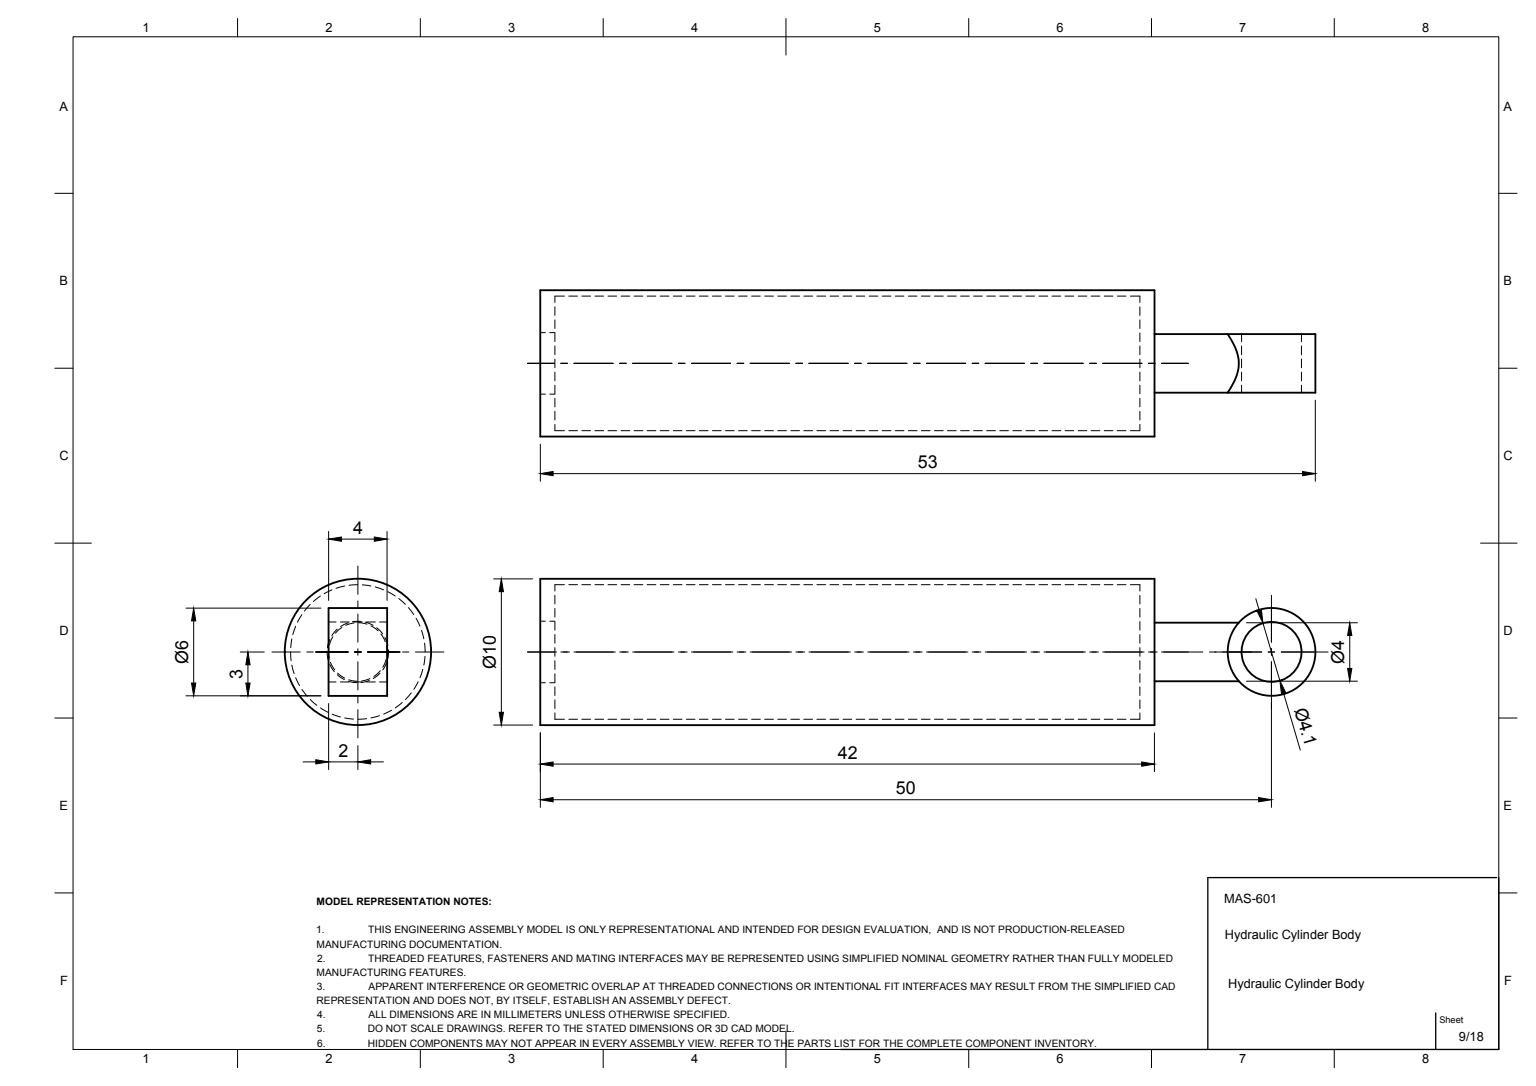
ISO-10303-21;
HEADER;
FILE_DESCRIPTION((''),'2;1');
FILE_NAME('Hydraulic Cylinder Body.step','2026-10-06T07:37:42+05:00',(''),(''),'','','');
FILE_SCHEMA (('AUTOMOTIVE_DESIGN { 1 0 10303 214 3 1 1 }'));
ENDSEC;
DATA;
#10=MECHANICAL_DESIGN_GEOMETRIC_PRESENTATION_REPRESENTATION('',(#377),#18757);
#343=SHAPE_REPRESENTATION_RELATIONSHIP('SRR','None',#18861,#360) ;
#360=ADVANCED_BREP_SHAPE_REPRESENTATION('',(#394),#18744) ;
#377=STYLED_ITEM('',(#18955),#394) ;
#394=MANIFOLD_SOLID_BREP('Hydraulic Cylinder Body',#9546) ;
#419=B_SPLINE_CURVE_WITH_KNOTS('',3,(#14585,#14586,#14587,#14588),
 .UNSPECIFIED.,.F.,.F.,(4,4),(0.941657228299601,0.974745769205032),
 .UNSPECIFIED.) ;
#420=B_SPLINE_CURVE_WITH_KNOTS('',3,(#14596,#14597,#14598,#14599,#14600,
#14601,#14602,#14603,#14604,#14605),.UNSPECIFIED.,.F.,.F.,(4,2,2,2,4),(0.313885742766534,
0.391923143756541,0.469960544746549,0.548866015139808,0.627771485533068),
 .UNSPECIFIED.) ;
#421=B_SPLINE_CURVE_WITH_KNOTS('',3,(#14606,#14607,#14608,#14609,#14610,
#14611,#14612,#14613,#14614,#14615),.UNSPECIFIED.,.F.,.F.,(4,2,2,2,4),(0.627771485533068,
0.706676955926327,0.785582426319586,0.863619827309594,0.941657228299601),
 .UNSPECIFIED.) ;
#422=B_SPLINE_CURVE_WITH_KNOTS('',3,(#14617,#14618,#14619,#14620,#14621,
#14622,#14623,#14624,#14625,#14626,#14627,#14628,#14629,#14630,#14631,#14632,
#14633,#14634,#14635),.UNSPECIFIED.,.F.,.F.,(4,2,2,2,3,2,2,2,4),(0.974745769205032,
1.01969462928961,1.09773203027962,1.17663750067288,1.25554297106614,1.33444844145939,
1.41335391185265,1.49139131284266,1.53634017292724),.UNSPECIFIED.) ;
#423=B_SPLINE_CURVE_WITH_KNOTS('',3,(#14667,#14668,#14669,#14670),
 .UNSPECIFIED.,.F.,.F.,(4,4),(1.53634017292724,1.56942871383267),
 .UNSPECIFIED.) ;
#561=CYLINDRICAL_SURFACE('',#10071,3.) ;
#562=CYLINDRICAL_SURFACE('',#10073,3.) ;
#563=CYLINDRICAL_SURFACE('',#10076,2.05) ;
#564=CYLINDRICAL_SURFACE('',#10081,4.6) ;
#565=CYLINDRICAL_SURFACE('',#10085,2.09999999999999) ;
#566=CYLINDRICAL_SURFACE('',#10089,4.99999999999999) ;
#567=CYLINDRICAL_SURFACE('',#10093,1.99999999999999) ;
#568=CYLINDRICAL_SURFACE('',#10094,3.) ;
#712=FACE_BOUND('',#1851,.T.) ;
#713=FACE_BOUND('',#1854,.T.) ;
#714=FACE_BOUND('',#1857,.T.) ;
#715=FACE_BOUND('',#1861,.T.) ;
#716=FACE_BOUND('',#1863,.T.) ;
#856=PLANE('',#10079) ;
#857=PLANE('',#10083) ;
#858=PLANE('',#10087) ;
#859=PLANE('',#10091) ;
#860=PLANE('',#10096) ;
#861=PLANE('',#10097) ;
#1265=FACE_OUTER_BOUND('',#1845,.T.) ;
#1266=FACE_OUTER_BOUND('',#1846,.T.) ;
#1267=FACE_OUTER_BOUND('',#1847,.T.) ;
#1268=FACE_OUTER_BOUND('',#1848,.T.) ;
#1269=FACE_OUTER_BOUND('',#1849,.T.) ;
#1270=FACE_OUTER_BOUND('',#1850,.T.) ;
#1271=FACE_OUTER_BOUND('',#1852,.T.) ;
#1272=FACE_OUTER_BOUND('',#1853,.T.) ;
#1273=FACE_OUTER_BOUND('',#1855,.T.) ;
#1274=FACE_OUTER_BOUND('',#1856,.T.) ;
#1275=FACE_OUTER_BOUND('',#1858,.T.) ;
#1276=FACE_OUTER_BOUND('',#1859,.T.) ;
#1277=FACE_OUTER_BOUND('',#1860,.T.) ;
#1278=FACE_OUTER_BOUND('',#1862,.T.) ;
#1845=EDGE_LOOP('',(#7257,#7258,#7259)) ;
#1846=EDGE_LOOP('',(#7260,#7261,#7262,#7263,#7264,#7265,#7266)) ;
#1847=EDGE_LOOP('',(#7267,#7268,#7269,#7270)) ;
#1848=EDGE_LOOP('',(#7271)) ;
#1849=EDGE_LOOP('',(#7272,#7273,#7274,#7275)) ;
#1850=EDGE_LOOP('',(#7276)) ;
#1851=EDGE_LOOP('',(#7277)) ;
#1852=EDGE_LOOP('',(#7278,#7279,#7280,#7281)) ;
#1853=EDGE_LOOP('',(#7282)) ;
#1854=EDGE_LOOP('',(#7283)) ;
#1855=EDGE_LOOP('',(#7284,#7285,#7286,#7287)) ;
#1856=EDGE_LOOP('',(#7288)) ;
#1857=EDGE_LOOP('',(#7289)) ;
#1858=EDGE_LOOP('',(#7290,#7291,#7292,#7293,#7294,#7295,#7296,#7297)) ;
#1859=EDGE_LOOP('',(#7298,#7299,#7300)) ;
#1860=EDGE_LOOP('',(#7301,#7302)) ;
#1861=EDGE_LOOP('',(#7303)) ;
#1862=EDGE_LOOP('',(#7304,#7305)) ;
#1863=EDGE_LOOP('',(#7306)) ;
#2538=LINE('',#14582,#3309) ;
#2539=LINE('',#14592,#3310) ;
#2540=LINE('',#14640,#3311) ;
#2541=LINE('',#14647,#3312) ;
#2542=LINE('',#14654,#3313) ;
#2543=LINE('',#14662,#3314) ;
#2544=LINE('',#14671,#3315) ;
#3309=VECTOR('',#11670,3.) ;
#3310=VECTOR('',#11675,3.) ;
#3311=VECTOR('',#11684,2.05) ;
#3312=VECTOR('',#11693,4.6) ;
#3313=VECTOR('',#11702,2.09999999999999) ;
#3314=VECTOR('',#11713,4.99999999999999) ;
#3315=VECTOR('',#11720,1.99999999999999) ;
#3915=CIRCLE('',#10072,3.) ;
#3916=CIRCLE('',#10074,3.) ;
#3917=CIRCLE('',#10075,3.) ;
#3918=CIRCLE('',#10077,2.05) ;
#3919=CIRCLE('',#10078,2.05) ;
#3920=CIRCLE('',#10080,4.6) ;
#3921=CIRCLE('',#10082,4.6) ;
#3922=CIRCLE('',#10084,2.1) ;
#3923=CIRCLE('',#10086,2.09999999999999) ;
#3924=CIRCLE('',#10088,4.99999999999999) ;
#3925=CIRCLE('',#10090,5.) ;
#3926=CIRCLE('',#10092,1.99999999999999) ;
#3927=CIRCLE('',#10095,3.) ;
#4450=VERTEX_POINT('',#14580) ;
#4451=VERTEX_POINT('',#14581) ;
#4452=VERTEX_POINT('',#14583) ;
#4453=VERTEX_POINT('',#14590) ;
#4454=VERTEX_POINT('',#14591) ;
#4455=VERTEX_POINT('',#14593) ;
#4456=VERTEX_POINT('',#14595) ;
#4457=VERTEX_POINT('',#14637) ;
#4458=VERTEX_POINT('',#14639) ;
#4459=VERTEX_POINT('',#14643) ;
#4460=VERTEX_POINT('',#14646) ;
#4461=VERTEX_POINT('',#14650) ;
#4462=VERTEX_POINT('',#14653) ;
#4463=VERTEX_POINT('',#14657) ;
#4464=VERTEX_POINT('',#14660) ;
#4465=VERTEX_POINT('',#14664) ;
#5475=EDGE_CURVE('',#4450,#4451,#2538,.T.) ;
#5476=EDGE_CURVE('',#4451,#4452,#3915,.T.) ;
#5477=EDGE_CURVE('',#4452,#4450,#419,.T.) ;
#5478=EDGE_CURVE('',#4453,#4454,#2539,.T.) ;
#5479=EDGE_CURVE('',#4455,#4453,#3916,.T.) ;
#5480=EDGE_CURVE('',#4455,#4456,#420,.T.) ;
#5481=EDGE_CURVE('',#4456,#4452,#421,.T.) ;
#5482=EDGE_CURVE('',#4452,#4451,#3917,.T.) ;
#5483=EDGE_CURVE('',#4450,#4454,#422,.T.) ;
#5484=EDGE_CURVE('',#4457,#4457,#3918,.T.) ;
#5485=EDGE_CURVE('',#4457,#4458,#2540,.T.) ;
#5486=EDGE_CURVE('',#4458,#4458,#3919,.T.) ;
#5487=EDGE_CURVE('',#4459,#4459,#3920,.T.) ;
#5488=EDGE_CURVE('',#4459,#4460,#2541,.T.) ;
#5489=EDGE_CURVE('',#4460,#4460,#3921,.T.) ;
#5490=EDGE_CURVE('',#4461,#4461,#3922,.T.) ;
#5491=EDGE_CURVE('',#4461,#4462,#2542,.T.) ;
#5492=EDGE_CURVE('',#4462,#4462,#3923,.T.) ;
#5493=EDGE_CURVE('',#4463,#4463,#3924,.T.) ;
#5494=EDGE_CURVE('',#4464,#4464,#3925,.T.) ;
#5495=EDGE_CURVE('',#4464,#4463,#2543,.T.) ;
#5496=EDGE_CURVE('',#4465,#4465,#3926,.T.) ;
#5497=EDGE_CURVE('',#4454,#4455,#423,.T.) ;
#5498=EDGE_CURVE('',#4456,#4465,#2544,.T.) ;
#5499=EDGE_CURVE('',#4453,#4455,#3927,.T.) ;
#7257=ORIENTED_EDGE('',*,*,#5475,.T.) ;
#7258=ORIENTED_EDGE('',*,*,#5476,.T.) ;
#7259=ORIENTED_EDGE('',*,*,#5477,.T.) ;
#7260=ORIENTED_EDGE('',*,*,#5478,.F.) ;
#7261=ORIENTED_EDGE('',*,*,#5479,.F.) ;
#7262=ORIENTED_EDGE('',*,*,#5480,.T.) ;
#7263=ORIENTED_EDGE('',*,*,#5481,.T.) ;
#7264=ORIENTED_EDGE('',*,*,#5482,.T.) ;
#7265=ORIENTED_EDGE('',*,*,#5475,.F.) ;
#7266=ORIENTED_EDGE('',*,*,#5483,.T.) ;
#7267=ORIENTED_EDGE('',*,*,#5484,.F.) ;
#7268=ORIENTED_EDGE('',*,*,#5485,.T.) ;
#7269=ORIENTED_EDGE('',*,*,#5486,.F.) ;
#7270=ORIENTED_EDGE('',*,*,#5485,.F.) ;
#7271=ORIENTED_EDGE('',*,*,#5487,.F.) ;
#7272=ORIENTED_EDGE('',*,*,#5487,.T.) ;
#7273=ORIENTED_EDGE('',*,*,#5488,.T.) ;
#7274=ORIENTED_EDGE('',*,*,#5489,.F.) ;
#7275=ORIENTED_EDGE('',*,*,#5488,.F.) ;
#7276=ORIENTED_EDGE('',*,*,#5489,.T.) ;
#7277=ORIENTED_EDGE('',*,*,#5490,.F.) ;
#7278=ORIENTED_EDGE('',*,*,#5490,.T.) ;
#7279=ORIENTED_EDGE('',*,*,#5491,.T.) ;
#7280=ORIENTED_EDGE('',*,*,#5492,.F.) ;
#7281=ORIENTED_EDGE('',*,*,#5491,.F.) ;
#7282=ORIENTED_EDGE('',*,*,#5493,.F.) ;
#7283=ORIENTED_EDGE('',*,*,#5492,.T.) ;
#7284=ORIENTED_EDGE('',*,*,#5494,.F.) ;
#7285=ORIENTED_EDGE('',*,*,#5495,.T.) ;
#7286=ORIENTED_EDGE('',*,*,#5493,.T.) ;
#7287=ORIENTED_EDGE('',*,*,#5495,.F.) ;
#7288=ORIENTED_EDGE('',*,*,#5494,.T.) ;
#7289=ORIENTED_EDGE('',*,*,#5496,.F.) ;
#7290=ORIENTED_EDGE('',*,*,#5480,.F.) ;
#7291=ORIENTED_EDGE('',*,*,#5497,.F.) ;
#7292=ORIENTED_EDGE('',*,*,#5483,.F.) ;
#7293=ORIENTED_EDGE('',*,*,#5477,.F.) ;
#7294=ORIENTED_EDGE('',*,*,#5481,.F.) ;
#7295=ORIENTED_EDGE('',*,*,#5498,.T.) ;
#7296=ORIENTED_EDGE('',*,*,#5496,.T.) ;
#7297=ORIENTED_EDGE('',*,*,#5498,.F.) ;
#7298=ORIENTED_EDGE('',*,*,#5478,.T.) ;
#7299=ORIENTED_EDGE('',*,*,#5497,.T.) ;
#7300=ORIENTED_EDGE('',*,*,#5499,.F.) ;
#7301=ORIENTED_EDGE('',*,*,#5479,.T.) ;
#7302=ORIENTED_EDGE('',*,*,#5499,.T.) ;
#7303=ORIENTED_EDGE('',*,*,#5486,.T.) ;
#7304=ORIENTED_EDGE('',*,*,#5482,.F.) ;
#7305=ORIENTED_EDGE('',*,*,#5476,.F.) ;
#7306=ORIENTED_EDGE('',*,*,#5484,.T.) ;
#9201=ADVANCED_FACE('',(#1265),#561,.T.) ;
#9202=ADVANCED_FACE('',(#1266),#562,.T.) ;
#9203=ADVANCED_FACE('',(#1267),#563,.F.) ;
#9204=ADVANCED_FACE('',(#1268),#856,.T.) ;
#9205=ADVANCED_FACE('',(#1269),#564,.F.) ;
#9206=ADVANCED_FACE('',(#1270,#712),#857,.T.) ;
#9207=ADVANCED_FACE('',(#1271),#565,.F.) ;
#9208=ADVANCED_FACE('',(#1272,#713),#858,.T.) ;
#9209=ADVANCED_FACE('',(#1273),#566,.T.) ;
#9210=ADVANCED_FACE('',(#1274,#714),#859,.T.) ;
#9211=ADVANCED_FACE('',(#1275),#567,.T.) ;
#9212=ADVANCED_FACE('',(#1276),#568,.T.) ;
#9213=ADVANCED_FACE('',(#1277,#715),#860,.T.) ;
#9214=ADVANCED_FACE('',(#1278,#716),#861,.F.) ;
#9546=CLOSED_SHELL('',(#9201,#9202,#9203,#9204,#9205,#9206,#9207,#9208,
#9209,#9210,#9211,#9212,#9213,#9214)) ;
#10070=AXIS2_PLACEMENT_3D('',#14578,#11666,#11667) ;
#10071=AXIS2_PLACEMENT_3D('',#14579,#11668,#11669) ;
#10072=AXIS2_PLACEMENT_3D('',#14584,#11671,#11672) ;
#10073=AXIS2_PLACEMENT_3D('',#14589,#11673,#11674) ;
#10074=AXIS2_PLACEMENT_3D('',#14594,#11676,#11677) ;
#10075=AXIS2_PLACEMENT_3D('',#14616,#11678,#11679) ;
#10076=AXIS2_PLACEMENT_3D('',#14636,#11680,#11681) ;
#10077=AXIS2_PLACEMENT_3D('',#14638,#11682,#11683) ;
#10078=AXIS2_PLACEMENT_3D('',#14641,#11685,#11686) ;
#10079=AXIS2_PLACEMENT_3D('',#14642,#11687,#11688) ;
#10080=AXIS2_PLACEMENT_3D('',#14644,#11689,#11690) ;
#10081=AXIS2_PLACEMENT_3D('',#14645,#11691,#11692) ;
#10082=AXIS2_PLACEMENT_3D('',#14648,#11694,#11695) ;
#10083=AXIS2_PLACEMENT_3D('',#14649,#11696,#11697) ;
#10084=AXIS2_PLACEMENT_3D('',#14651,#11698,#11699) ;
#10085=AXIS2_PLACEMENT_3D('',#14652,#11700,#11701) ;
#10086=AXIS2_PLACEMENT_3D('',#14655,#11703,#11704) ;
#10087=AXIS2_PLACEMENT_3D('',#14656,#11705,#11706) ;
#10088=AXIS2_PLACEMENT_3D('',#14658,#11707,#11708) ;
#10089=AXIS2_PLACEMENT_3D('',#14659,#11709,#11710) ;
#10090=AXIS2_PLACEMENT_3D('',#14661,#11711,#11712) ;
#10091=AXIS2_PLACEMENT_3D('',#14663,#11714,#11715) ;
#10092=AXIS2_PLACEMENT_3D('',#14665,#11716,#11717) ;
#10093=AXIS2_PLACEMENT_3D('',#14666,#11718,#11719) ;
#10094=AXIS2_PLACEMENT_3D('',#14672,#11721,#11722) ;
#10095=AXIS2_PLACEMENT_3D('',#14673,#11723,#11724) ;
#10096=AXIS2_PLACEMENT_3D('',#14674,#11725,#11726) ;
#10097=AXIS2_PLACEMENT_3D('',#14675,#11727,#11728) ;
#11666=DIRECTION('axis',(0.,0.,1.)) ;
#11667=DIRECTION('refdir',(1.,0.,0.)) ;
#11668=DIRECTION('center_axis',(0.,1.,0.)) ;
#11669=DIRECTION('ref_axis',(1.,0.,0.)) ;
#11670=DIRECTION('',(0.,-1.,0.)) ;
#11671=DIRECTION('center_axis',(0.,1.,0.)) ;
#11672=DIRECTION('ref_axis',(1.,0.,0.)) ;
#11673=DIRECTION('center_axis',(0.,1.,0.)) ;
#11674=DIRECTION('ref_axis',(1.,0.,0.)) ;
#11675=DIRECTION('',(0.,-1.,0.)) ;
#11676=DIRECTION('center_axis',(0.,1.,0.)) ;
#11677=DIRECTION('ref_axis',(1.,0.,0.)) ;
#11678=DIRECTION('center_axis',(0.,1.,0.)) ;
#11679=DIRECTION('ref_axis',(1.,0.,0.)) ;
#11680=DIRECTION('center_axis',(0.,1.,0.)) ;
#11681=DIRECTION('ref_axis',(1.,0.,0.)) ;
#11682=DIRECTION('center_axis',(0.,1.,0.)) ;
#11683=DIRECTION('ref_axis',(1.,0.,0.)) ;
#11684=DIRECTION('',(0.,1.,0.)) ;
#11685=DIRECTION('center_axis',(0.,-1.,0.)) ;
#11686=DIRECTION('ref_axis',(1.,0.,0.)) ;
#11687=DIRECTION('center_axis',(-0.993765553407216,0.,0.11149002135281)) ;
#11688=DIRECTION('ref_axis',(0.11149002135281,0.,0.993765553407216)) ;
#11689=DIRECTION('center_axis',(0.993765553407216,0.,-0.11149002135281)) ;
#11690=DIRECTION('ref_axis',(0.11149002135281,0.,0.993765553407216)) ;
#11691=DIRECTION('center_axis',(0.993765553407216,0.,-0.11149002135281)) ;
#11692=DIRECTION('ref_axis',(-0.111490021352808,0.,-0.993765553407216)) ;
#11693=DIRECTION('',(-0.993765553407216,0.,0.11149002135281)) ;
#11694=DIRECTION('center_axis',(0.993765553407216,0.,-0.11149002135281)) ;
#11695=DIRECTION('ref_axis',(0.11149002135281,0.,0.993765553407216)) ;
#11696=DIRECTION('center_axis',(0.993765553407216,0.,-0.11149002135281)) ;
#11697=DIRECTION('ref_axis',(-0.11149002135281,0.,-0.993765553407216)) ;
#11698=DIRECTION('center_axis',(0.993765553407216,0.,-0.11149002135281)) ;
#11699=DIRECTION('ref_axis',(0.11149002135281,0.,0.993765553407216)) ;
#11700=DIRECTION('center_axis',(0.993765553407216,0.,-0.11149002135281)) ;
#11701=DIRECTION('ref_axis',(-0.111490021352808,0.,-0.993765553407216)) ;
#11702=DIRECTION('',(-0.993765553407216,0.,0.11149002135281)) ;
#11703=DIRECTION('center_axis',(0.993765553407216,0.,-0.11149002135281)) ;
#11704=DIRECTION('ref_axis',(0.11149002135281,0.,0.993765553407216)) ;
#11705=DIRECTION('center_axis',(-0.993765553407216,0.,0.11149002135281)) ;
#11706=DIRECTION('ref_axis',(0.11149002135281,0.,0.993765553407216)) ;
#11707=DIRECTION('center_axis',(0.993765553407216,0.,-0.11149002135281)) ;
#11708=DIRECTION('ref_axis',(0.11149002135281,0.,0.993765553407216)) ;
#11709=DIRECTION('center_axis',(0.993765553407216,0.,-0.11149002135281)) ;
#11710=DIRECTION('ref_axis',(-0.111490021352808,0.,-0.993765553407216)) ;
#11711=DIRECTION('center_axis',(0.993765553407216,0.,-0.11149002135281)) ;
#11712=DIRECTION('ref_axis',(0.11149002135281,0.,0.993765553407216)) ;
#11713=DIRECTION('',(-0.993765553407216,0.,0.11149002135281)) ;
#11714=DIRECTION('center_axis',(0.993765553407216,0.,-0.11149002135281)) ;
#11715=DIRECTION('ref_axis',(-0.11149002135281,0.,-0.993765553407216)) ;
#11716=DIRECTION('center_axis',(0.993765553407216,0.,-0.11149002135281)) ;
#11717=DIRECTION('ref_axis',(0.11149002135281,0.,0.993765553407216)) ;
#11718=DIRECTION('center_axis',(0.993765553407216,0.,-0.11149002135281)) ;
#11719=DIRECTION('ref_axis',(-0.111490021352808,0.,-0.993765553407216)) ;
#11720=DIRECTION('',(-0.993765553407216,0.,0.11149002135281)) ;
#11721=DIRECTION('center_axis',(0.,1.,0.)) ;
#11722=DIRECTION('ref_axis',(1.,0.,0.)) ;
#11723=DIRECTION('center_axis',(0.,1.,0.)) ;
#11724=DIRECTION('ref_axis',(1.,0.,0.)) ;
#11725=DIRECTION('center_axis',(0.,1.,0.)) ;
#11726=DIRECTION('ref_axis',(1.,0.,0.)) ;
#11727=DIRECTION('center_axis',(0.,1.,0.)) ;
#11728=DIRECTION('ref_axis',(1.,0.,0.)) ;
#14578=CARTESIAN_POINT('',(0.,0.,0.)) ;
#14579=CARTESIAN_POINT('Origin',(77.,-2.,35.)) ;
#14580=CARTESIAN_POINT('',(74.,-1.97183411479483,35.000000000015)) ;
#14581=CARTESIAN_POINT('',(74.,-2.,35.)) ;
#14582=CARTESIAN_POINT('',(74.,-2.,35.)) ;
#14583=CARTESIAN_POINT('',(74.0187033397783,-2.,35.3344700640584)) ;
#14584=CARTESIAN_POINT('Origin',(77.,-2.,35.)) ;
#14585=CARTESIAN_POINT('Ctrl Pts',(74.0187033397784,-1.99999999999999,35.3344700640584)) ;
#14586=CARTESIAN_POINT('Ctrl Pts',(74.0064065326714,-1.99999999999999,35.224862556844)) ;
#14587=CARTESIAN_POINT('Ctrl Pts',(74.0000000000011,-1.99077077040239,35.1123394944064)) ;
#14588=CARTESIAN_POINT('Ctrl Pts',(74.,-1.97183411479483,35.0000000000301)) ;
#14589=CARTESIAN_POINT('Origin',(77.,-2.,35.)) ;
#14590=CARTESIAN_POINT('',(74.,2.,35.)) ;
#14591=CARTESIAN_POINT('',(74.,1.97183411479483,35.000000000015)) ;
#14592=CARTESIAN_POINT('',(74.,-2.,35.)) ;
#14593=CARTESIAN_POINT('',(74.0187033397783,2.,35.3344700640584)) ;
#14594=CARTESIAN_POINT('Origin',(77.,2.,35.)) ;
#14595=CARTESIAN_POINT('',(75.0008527115894,-2.4492935982947E-16,37.2368303733722)) ;
#14596=CARTESIAN_POINT('Ctrl Pts',(74.0187033397784,1.99999999999999,35.3344700640584)) ;
#14597=CARTESIAN_POINT('Ctrl Pts',(74.0477046447873,1.99999999999999,35.5929730006627)) ;
#14598=CARTESIAN_POINT('Ctrl Pts',(74.1144354069026,1.94624453140306,35.8591102084627)) ;
#14599=CARTESIAN_POINT('Ctrl Pts',(74.3000163132069,1.73918232877706,36.3321566427019)) ;
#14600=CARTESIAN_POINT('Ctrl Pts',(74.4178370345461,1.58626985902425,36.5396414824713)) ;
#14601=CARTESIAN_POINT('Ctrl Pts',(74.6402213681462,1.24024335258715,36.862889628107)) ;
#14602=CARTESIAN_POINT('Ctrl Pts',(74.7617847795615,1.02133350899655,37.0018504709194)) ;
#14603=CARTESIAN_POINT('Ctrl Pts',(74.943978655708,0.533317960206907,37.1885590945277)) ;
#14604=CARTESIAN_POINT('Ctrl Pts',(75.0008527115894,0.263018234644198,37.2368303733722)) ;
#14605=CARTESIAN_POINT('Ctrl Pts',(75.0008527115894,5.55111512312578E-16,
37.2368303733722)) ;
#14606=CARTESIAN_POINT('Ctrl Pts',(75.0008527115894,-1.38777878078145E-16,
37.2368303733722)) ;
#14607=CARTESIAN_POINT('Ctrl Pts',(75.0008527115894,-0.263018234644197,
37.2368303733722)) ;
#14608=CARTESIAN_POINT('Ctrl Pts',(74.943978655708,-0.533317960206906,37.1885590945277)) ;
#14609=CARTESIAN_POINT('Ctrl Pts',(74.7617847795615,-1.02133350899655,37.0018504709194)) ;
#14610=CARTESIAN_POINT('Ctrl Pts',(74.6402213681462,-1.24024335258715,36.862889628107)) ;
#14611=CARTESIAN_POINT('Ctrl Pts',(74.4178370345462,-1.58626985902425,36.5396414824713)) ;
#14612=CARTESIAN_POINT('Ctrl Pts',(74.3000163132069,-1.73918232877706,36.3321566427019)) ;
#14613=CARTESIAN_POINT('Ctrl Pts',(74.1144354069026,-1.94624453140306,35.8591102084627)) ;
#14614=CARTESIAN_POINT('Ctrl Pts',(74.0477046447873,-1.99999999999999,35.5929730006628)) ;
#14615=CARTESIAN_POINT('Ctrl Pts',(74.0187033397784,-1.99999999999999,35.3344700640584)) ;
#14616=CARTESIAN_POINT('Origin',(77.,-2.,35.)) ;
#14617=CARTESIAN_POINT('Ctrl Pts',(74.,-1.97183411479483,35.0000000000301)) ;
#14618=CARTESIAN_POINT('Ctrl Pts',(73.9999999999985,-1.94610976853832,34.8473933248331)) ;
#14619=CARTESIAN_POINT('Ctrl Pts',(74.0119436372818,-1.90234643847172,34.6951462661377)) ;
#14620=CARTESIAN_POINT('Ctrl Pts',(74.0719456039354,-1.73918232877706,34.2992499137851)) ;
#14621=CARTESIAN_POINT('Ctrl Pts',(74.1408607543884,-1.58626985902425,34.0708152772934)) ;
#14622=CARTESIAN_POINT('Ctrl Pts',(74.2860880828058,-1.24024335258715,33.706324977603)) ;
#14623=CARTESIAN_POINT('Ctrl Pts',(74.3738371045158,-1.02133350899655,33.5438814858313)) ;
#14624=CARTESIAN_POINT('Ctrl Pts',(74.5101288893078,-0.533317960206906,
33.3214421277285)) ;
#14625=CARTESIAN_POINT('Ctrl Pts',(74.5548926261781,-0.263018234644197,
33.2617681597434)) ;
#14626=CARTESIAN_POINT('Ctrl Pts',(74.5548926261781,0.,33.2617681597434)) ;
#14627=CARTESIAN_POINT('Ctrl Pts',(74.5548926261781,0.263018234644197,33.2617681597434)) ;
#14628=CARTESIAN_POINT('Ctrl Pts',(74.5101288893078,0.533317960206908,33.3214421277285)) ;
#14629=CARTESIAN_POINT('Ctrl Pts',(74.3738371045158,1.02133350899655,33.5438814858313)) ;
#14630=CARTESIAN_POINT('Ctrl Pts',(74.2860880828058,1.24024335258715,33.706324977603)) ;
#14631=CARTESIAN_POINT('Ctrl Pts',(74.1408607543884,1.58626985902425,34.0708152772934)) ;
#14632=CARTESIAN_POINT('Ctrl Pts',(74.0719456039354,1.73918232877707,34.2992499137851)) ;
#14633=CARTESIAN_POINT('Ctrl Pts',(74.0119436372818,1.90234643847172,34.6951462661377)) ;
#14634=CARTESIAN_POINT('Ctrl Pts',(73.9999999999985,1.94610976853832,34.8473933248331)) ;
#14635=CARTESIAN_POINT('Ctrl Pts',(74.,1.97183411479483,35.0000000000301)) ;
#14636=CARTESIAN_POINT('Origin',(77.,-2.5,35.)) ;
#14637=CARTESIAN_POINT('',(74.95,-2.,35.)) ;
#14638=CARTESIAN_POINT('Origin',(77.,-2.,35.)) ;
#14639=CARTESIAN_POINT('',(74.95,2.,35.)) ;
#14640=CARTESIAN_POINT('',(74.95,-2.5,35.)) ;
#14641=CARTESIAN_POINT('Origin',(77.,2.,35.)) ;
#14642=CARTESIAN_POINT('Origin',(67.5432559211121,0.,31.4320886465021)) ;
#14643=CARTESIAN_POINT('',(68.568964117558,-5.63337527607782E-16,40.5747317378485)) ;
#14644=CARTESIAN_POINT('Origin',(68.0561100193351,0.,36.0034101921753)) ;
#14645=CARTESIAN_POINT('Origin',(48.1807989511907,0.,38.2332106192315)) ;
#14646=CARTESIAN_POINT('',(28.8183419812693,-5.63337527607782E-16,45.0343325919609)) ;
#14647=CARTESIAN_POINT('',(48.6936530494136,-5.63337527607782E-16,42.8045321649047)) ;
#14648=CARTESIAN_POINT('Origin',(28.3054878830464,0.,40.4630110462877)) ;
#14649=CARTESIAN_POINT('Origin',(28.0713588382055,0.,38.3761033841325)) ;
#14650=CARTESIAN_POINT('',(28.5396169278873,-2.57175827820943E-16,42.5499187084428)) ;
#14651=CARTESIAN_POINT('Origin',(28.3054878830464,0.,40.4630110462877)) ;
#14652=CARTESIAN_POINT('Origin',(27.8086051063428,0.,40.5187560569641)) ;
#14653=CARTESIAN_POINT('',(27.5458513744801,-2.57175827820943E-16,42.6614087297956)) ;
#14654=CARTESIAN_POINT('',(28.0427341511837,-2.57175827820943E-16,42.6056637191192)) ;
#14655=CARTESIAN_POINT('Origin',(27.3117223296392,0.,40.5745010676405)) ;
#14656=CARTESIAN_POINT('Origin',(26.7542722228752,0.,35.6056733006044)) ;
#14657=CARTESIAN_POINT('',(27.8691724364032,-6.12323399573676E-16,45.5433288346766)) ;
#14658=CARTESIAN_POINT('Origin',(27.3117223296392,0.,40.5745010676405)) ;
#14659=CARTESIAN_POINT('Origin',(48.1807989511907,0.,38.2332106192315)) ;
#14660=CARTESIAN_POINT('',(69.6073256795063,-6.12323399573676E-16,40.8607479378586)) ;
#14661=CARTESIAN_POINT('Origin',(69.0498755727423,0.,35.8919201708225)) ;
#14662=CARTESIAN_POINT('',(48.7382490579548,-6.12323399573676E-16,43.2020383862676)) ;
#14663=CARTESIAN_POINT('Origin',(68.8268955300367,0.,33.9043890640081)) ;
#14664=CARTESIAN_POINT('',(69.2728556154479,-2.4492935982947E-16,37.8794512776369)) ;
#14665=CARTESIAN_POINT('Origin',(69.0498755727423,0.,35.8919201708225)) ;
#14666=CARTESIAN_POINT('Origin',(72.0311722329639,0.,35.557450106764)) ;
#14667=CARTESIAN_POINT('Ctrl Pts',(74.,1.97183411479483,35.0000000000301)) ;
#14668=CARTESIAN_POINT('Ctrl Pts',(74.0000000000011,1.99077077040239,35.1123394944064)) ;
#14669=CARTESIAN_POINT('Ctrl Pts',(74.0064065326714,1.99999999999999,35.224862556844)) ;
#14670=CARTESIAN_POINT('Ctrl Pts',(74.0187033397784,1.99999999999999,35.3344700640584)) ;
#14671=CARTESIAN_POINT('',(72.2541522756695,-2.4492935982947E-16,37.5449812135785)) ;
#14672=CARTESIAN_POINT('Origin',(77.,-2.,35.)) ;
#14673=CARTESIAN_POINT('Origin',(77.,2.,35.)) ;
#14674=CARTESIAN_POINT('Origin',(77.,2.,35.)) ;
#14675=CARTESIAN_POINT('Origin',(77.,-2.,35.)) ;
#18725=UNCERTAINTY_MEASURE_WITH_UNIT(LENGTH_MEASURE(0.01),#18758,
'DISTANCE_ACCURACY_VALUE',
'Maximum model space distance between geometric entities at asserted c
onnectivities') ;
#18738=UNCERTAINTY_MEASURE_WITH_UNIT(LENGTH_MEASURE(0.01),#18758,
'DISTANCE_ACCURACY_VALUE',
'Maximum model space distance between geometric entities at asserted c
onnectivities') ;
#18744=(
GEOMETRIC_REPRESENTATION_CONTEXT(3)
GLOBAL_UNCERTAINTY_ASSIGNED_CONTEXT((#18725))
GLOBAL_UNIT_ASSIGNED_CONTEXT((#18758,#18760,#18761))
REPRESENTATION_CONTEXT('','3D')
) ;
#18757=(
GEOMETRIC_REPRESENTATION_CONTEXT(3)
GLOBAL_UNCERTAINTY_ASSIGNED_CONTEXT((#18738))
GLOBAL_UNIT_ASSIGNED_CONTEXT((#18758,#18760,#18761))
REPRESENTATION_CONTEXT('','3D')
) ;
#18758=(
LENGTH_UNIT()
NAMED_UNIT(*)
SI_UNIT(.MILLI.,.METRE.)
) ;
#18760=(
NAMED_UNIT(*)
PLANE_ANGLE_UNIT()
SI_UNIT($,.RADIAN.)
) ;
#18761=(
NAMED_UNIT(*)
SI_UNIT($,.STERADIAN.)
SOLID_ANGLE_UNIT()
) ;
#18767=SHAPE_DEFINITION_REPRESENTATION(#18785,#18861) ;
#18785=PRODUCT_DEFINITION_SHAPE('',$,#18880) ;
#18861=SHAPE_REPRESENTATION('',(#10070),#18744) ;
#18874=PRODUCT_DEFINITION_CONTEXT('part definition',#18930,'design') ;
#18880=PRODUCT_DEFINITION('Hydraulic Cylinder Body',
'Hydraulic Cylinder Body',#18898,#18874) ;
#18898=PRODUCT_DEFINITION_FORMATION('',$,#18937) ;
#18930=APPLICATION_CONTEXT(
'Core Data for Automotive Mechanical Design Process') ;
#18931=PRODUCT_CONTEXT('part definition',#18930,'mechanical') ;
#18937=PRODUCT('Hydraulic Cylinder Body','Hydraulic Cylinder Body',$,(#18931)) ;
#18955=PRESENTATION_STYLE_ASSIGNMENT((#18973)) ;
#18973=SURFACE_STYLE_USAGE(.BOTH.,#18991) ;
#18991=SURFACE_SIDE_STYLE('',(#19009)) ;
#19009=SURFACE_STYLE_FILL_AREA(#19027) ;
#19027=FILL_AREA_STYLE(
'MAS-253 Metallic Sheet - Hydraulic Cylinder Body',(#19045)) ;
#19045=FILL_AREA_STYLE_COLOUR(
'MAS-253 Metallic Sheet - Hydraulic Cylinder Body',#19063) ;
#19063=COLOUR_RGB('MAS-253 Metallic Sheet - Hydraulic Cylinder Body', 0.08235294, 0.09019608, 0.10196078) ;
ENDSEC;
END-ISO-10303-21;
